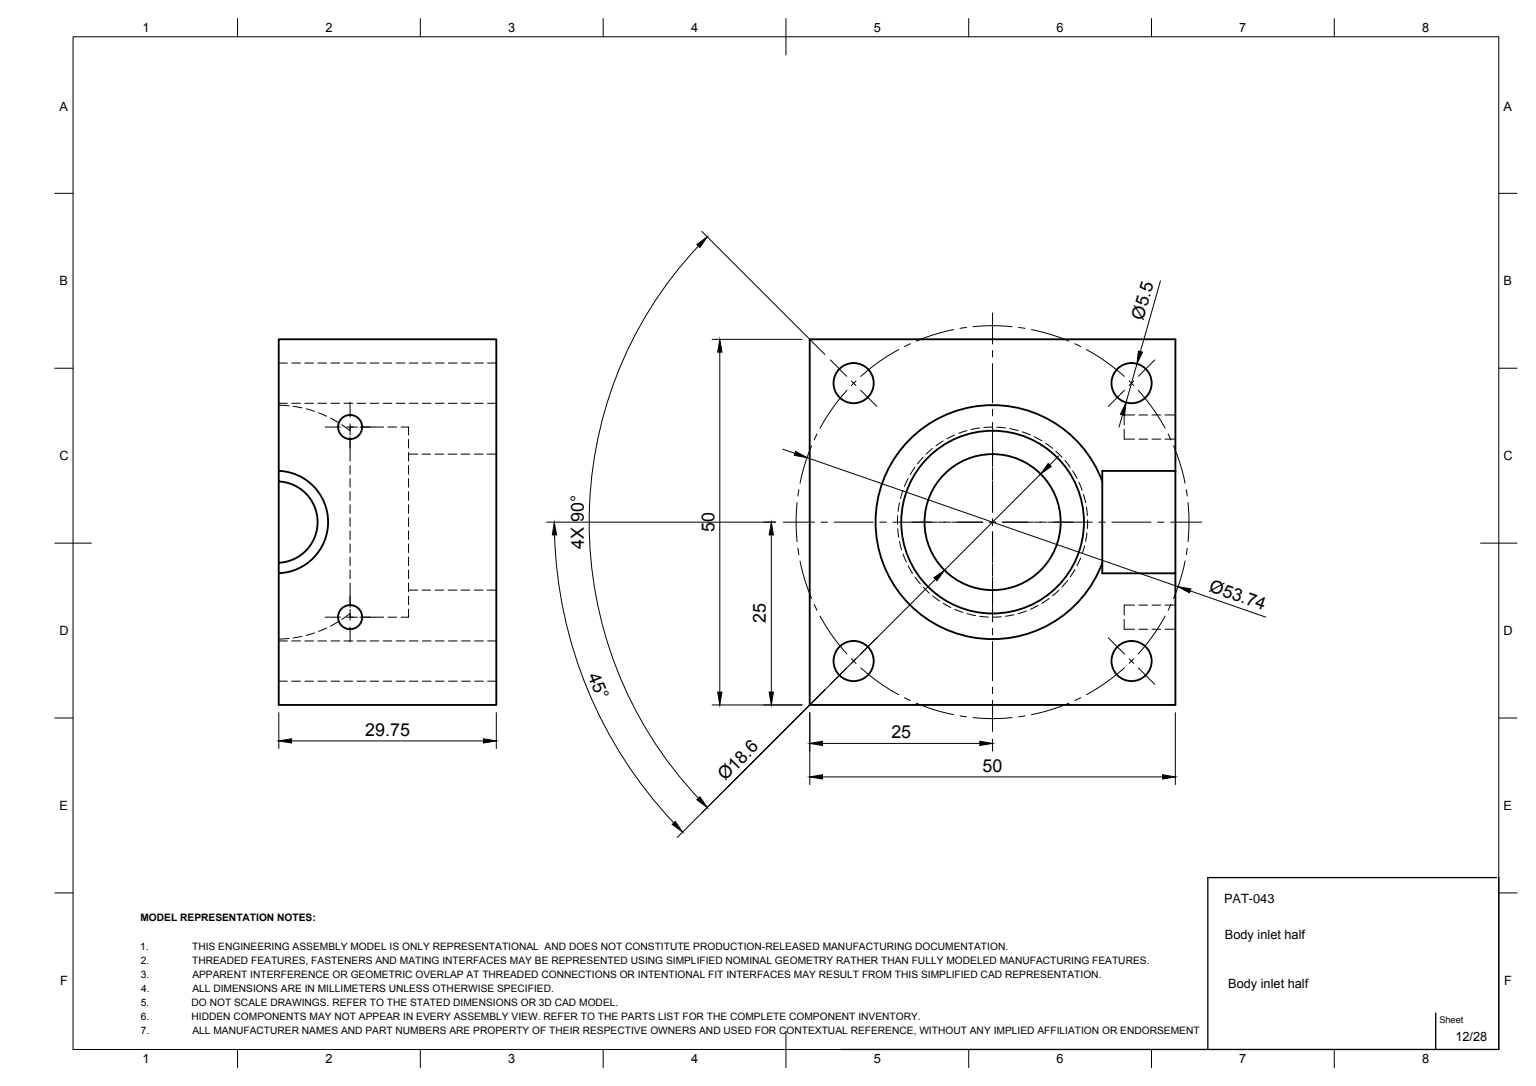
ISO-10303-21;
HEADER;
/* Generated by software containing ST-Developer
 * from STEP Tools, Inc. (www.steptools.com) 
 */

FILE_DESCRIPTION(
/* description */ ('Four-valve pipe header'),
/* implementation_level */ '2;1');

FILE_NAME(
/* name */ 'Body inlet half.step',
/* time_stamp */ '2026-10-29T16:56:19-07:00',
/* author */ (''),
/* organization */ (''),
/* preprocessor_version */ 'ST-DEVELOPER v20.2',
/* originating_system */ 'Autodesk Translation Framework v15.17.0.0',
/* authorisation */ '');

FILE_SCHEMA (('AUTOMOTIVE_DESIGN { 1 0 10303 214 3 1 1 }'));
ENDSEC;

DATA;
#10=MECHANICAL_DESIGN_GEOMETRIC_PRESENTATION_REPRESENTATION('',(#338),#10119);
#242=SPHERICAL_SURFACE('',#6142,1.6);
#286=SHAPE_REPRESENTATION_RELATIONSHIP('SRR','None',#10248,#312);
#312=ADVANCED_BREP_SHAPE_REPRESENTATION('',(#364),#10097);
#338=STYLED_ITEM('',(#10449),#364);
#364=MANIFOLD_SOLID_BREP('Body1',#5584);
#456=FACE_BOUND('',#1223,.T.);
#457=FACE_BOUND('',#1224,.T.);
#458=FACE_BOUND('',#1228,.T.);
#459=FACE_BOUND('',#1230,.T.);
#460=FACE_BOUND('',#1232,.T.);
#461=FACE_BOUND('',#1234,.T.);
#462=FACE_BOUND('',#1235,.T.);
#463=FACE_BOUND('',#1236,.T.);
#464=FACE_BOUND('',#1237,.T.);
#465=FACE_BOUND('',#1240,.T.);
#466=FACE_BOUND('',#1241,.T.);
#467=FACE_BOUND('',#1242,.T.);
#468=FACE_BOUND('',#1243,.T.);
#469=FACE_BOUND('',#1244,.T.);
#597=PLANE('',#6110);
#598=PLANE('',#6114);
#599=PLANE('',#6130);
#600=PLANE('',#6132);
#601=PLANE('',#6139);
#602=PLANE('',#6141);
#603=PLANE('',#6144);
#604=PLANE('',#6145);
#605=PLANE('',#6146);
#606=PLANE('',#6147);
#607=PLANE('',#6148);
#850=FACE_OUTER_BOUND('',#1212,.T.);
#851=FACE_OUTER_BOUND('',#1213,.T.);
#852=FACE_OUTER_BOUND('',#1214,.T.);
#853=FACE_OUTER_BOUND('',#1215,.T.);
#854=FACE_OUTER_BOUND('',#1216,.T.);
#855=FACE_OUTER_BOUND('',#1217,.T.);
#856=FACE_OUTER_BOUND('',#1218,.T.);
#857=FACE_OUTER_BOUND('',#1219,.T.);
#858=FACE_OUTER_BOUND('',#1220,.T.);
#859=FACE_OUTER_BOUND('',#1221,.T.);
#860=FACE_OUTER_BOUND('',#1222,.T.);
#861=FACE_OUTER_BOUND('',#1225,.T.);
#862=FACE_OUTER_BOUND('',#1226,.T.);
#863=FACE_OUTER_BOUND('',#1227,.T.);
#864=FACE_OUTER_BOUND('',#1229,.T.);
#865=FACE_OUTER_BOUND('',#1231,.T.);
#866=FACE_OUTER_BOUND('',#1233,.T.);
#867=FACE_OUTER_BOUND('',#1238,.T.);
#868=FACE_OUTER_BOUND('',#1239,.T.);
#869=FACE_OUTER_BOUND('',#1245,.T.);
#870=FACE_OUTER_BOUND('',#1246,.T.);
#1212=EDGE_LOOP('',(#4215,#4216,#4217,#4218));
#1213=EDGE_LOOP('',(#4219));
#1214=EDGE_LOOP('',(#4220,#4221,#4222,#4223));
#1215=EDGE_LOOP('',(#4224));
#1216=EDGE_LOOP('',(#4225,#4226,#4227,#4228));
#1217=EDGE_LOOP('',(#4229,#4230,#4231,#4232));
#1218=EDGE_LOOP('',(#4233,#4234,#4235,#4236));
#1219=EDGE_LOOP('',(#4237,#4238,#4239,#4240));
#1220=EDGE_LOOP('',(#4241,#4242,#4243,#4244));
#1221=EDGE_LOOP('',(#4245,#4246,#4247,#4248));
#1222=EDGE_LOOP('',(#4249,#4250,#4251,#4252,#4253,#4254));
#1223=EDGE_LOOP('',(#4255));
#1224=EDGE_LOOP('',(#4256));
#1225=EDGE_LOOP('',(#4257,#4258,#4259,#4260));
#1226=EDGE_LOOP('',(#4261,#4262,#4263,#4264));
#1227=EDGE_LOOP('',(#4265));
#1228=EDGE_LOOP('',(#4266));
#1229=EDGE_LOOP('',(#4267));
#1230=EDGE_LOOP('',(#4268));
#1231=EDGE_LOOP('',(#4269,#4270));
#1232=EDGE_LOOP('',(#4271));
#1233=EDGE_LOOP('',(#4272,#4273,#4274,#4275,#4276,#4277,#4278,#4279,#4280,
#4281));
#1234=EDGE_LOOP('',(#4282));
#1235=EDGE_LOOP('',(#4283));
#1236=EDGE_LOOP('',(#4284));
#1237=EDGE_LOOP('',(#4285));
#1238=EDGE_LOOP('',(#4286,#4287,#4288,#4289));
#1239=EDGE_LOOP('',(#4290,#4291,#4292,#4293));
#1240=EDGE_LOOP('',(#4294));
#1241=EDGE_LOOP('',(#4295));
#1242=EDGE_LOOP('',(#4296));
#1243=EDGE_LOOP('',(#4297));
#1244=EDGE_LOOP('',(#4298));
#1245=EDGE_LOOP('',(#4299,#4300,#4301,#4302));
#1246=EDGE_LOOP('',(#4303,#4304,#4305,#4306));
#1639=LINE('',#8960,#2057);
#1640=LINE('',#8967,#2058);
#1641=LINE('',#8974,#2059);
#1642=LINE('',#8980,#2060);
#1643=LINE('',#8986,#2061);
#1644=LINE('',#8992,#2062);
#1645=LINE('',#8997,#2063);
#1646=LINE('',#9001,#2064);
#1647=LINE('',#9005,#2065);
#1648=LINE('',#9008,#2066);
#1649=LINE('',#9011,#2067);
#1650=LINE('',#9013,#2068);
#1651=LINE('',#9015,#2069);
#1652=LINE('',#9017,#2070);
#1653=LINE('',#9018,#2071);
#1654=LINE('',#9023,#2072);
#1655=LINE('',#9029,#2073);
#1656=LINE('',#9039,#2074);
#1657=LINE('',#9041,#2075);
#1658=LINE('',#9042,#2076);
#1659=LINE('',#9045,#2077);
#1660=LINE('',#9046,#2078);
#1661=LINE('',#9049,#2079);
#1662=LINE('',#9050,#2080);
#1663=LINE('',#9052,#2081);
#2057=VECTOR('',#7116,0.165);
#2058=VECTOR('',#7125,0.165);
#2059=VECTOR('',#7134,0.275);
#2060=VECTOR('',#7141,0.275);
#2061=VECTOR('',#7148,0.275);
#2062=VECTOR('',#7155,0.275);
#2063=VECTOR('',#7160,1.);
#2064=VECTOR('',#7163,1.);
#2065=VECTOR('',#7168,1.);
#2066=VECTOR('',#7171,1.);
#2067=VECTOR('',#7174,1.);
#2068=VECTOR('',#7175,1.);
#2069=VECTOR('',#7176,1.);
#2070=VECTOR('',#7177,1.);
#2071=VECTOR('',#7178,1.);
#2072=VECTOR('',#7183,0.93);
#2073=VECTOR('',#7190,1.3);
#2074=VECTOR('',#7205,1.);
#2075=VECTOR('',#7206,1.);
#2076=VECTOR('',#7207,1.);
#2077=VECTOR('',#7210,1.);
#2078=VECTOR('',#7211,1.);
#2079=VECTOR('',#7214,1.);
#2080=VECTOR('',#7215,1.);
#2081=VECTOR('',#7218,1.);
#2424=CIRCLE('',#6108,0.165);
#2425=CIRCLE('',#6109,0.165);
#2426=CIRCLE('',#6112,0.165);
#2427=CIRCLE('',#6113,0.165);
#2428=CIRCLE('',#6116,0.275);
#2429=CIRCLE('',#6117,0.275);
#2430=CIRCLE('',#6119,0.275);
#2431=CIRCLE('',#6120,0.275);
#2432=CIRCLE('',#6122,0.275);
#2433=CIRCLE('',#6123,0.275);
#2434=CIRCLE('',#6125,0.275);
#2435=CIRCLE('',#6126,0.275);
#2436=CIRCLE('',#6128,0.7);
#2437=CIRCLE('',#6129,0.7);
#2438=CIRCLE('',#6131,0.556776436283003);
#2439=CIRCLE('',#6134,0.93);
#2440=CIRCLE('',#6135,0.93);
#2441=CIRCLE('',#6137,1.3);
#2442=CIRCLE('',#6138,1.3);
#2443=CIRCLE('',#6140,1.24899959967968);
#2444=CIRCLE('',#6143,1.59980467557762);
#2732=VERTEX_POINT('',#8957);
#2733=VERTEX_POINT('',#8959);
#2734=VERTEX_POINT('',#8964);
#2735=VERTEX_POINT('',#8966);
#2736=VERTEX_POINT('',#8971);
#2737=VERTEX_POINT('',#8973);
#2738=VERTEX_POINT('',#8977);
#2739=VERTEX_POINT('',#8979);
#2740=VERTEX_POINT('',#8983);
#2741=VERTEX_POINT('',#8985);
#2742=VERTEX_POINT('',#8989);
#2743=VERTEX_POINT('',#8991);
#2744=VERTEX_POINT('',#8995);
#2745=VERTEX_POINT('',#8996);
#2746=VERTEX_POINT('',#8998);
#2747=VERTEX_POINT('',#9000);
#2748=VERTEX_POINT('',#9004);
#2749=VERTEX_POINT('',#9006);
#2750=VERTEX_POINT('',#9010);
#2751=VERTEX_POINT('',#9012);
#2752=VERTEX_POINT('',#9014);
#2753=VERTEX_POINT('',#9016);
#2754=VERTEX_POINT('',#9020);
#2755=VERTEX_POINT('',#9022);
#2756=VERTEX_POINT('',#9026);
#2757=VERTEX_POINT('',#9028);
#2758=VERTEX_POINT('',#9032);
#2759=VERTEX_POINT('',#9038);
#2760=VERTEX_POINT('',#9040);
#2761=VERTEX_POINT('',#9044);
#2762=VERTEX_POINT('',#9048);
#3274=EDGE_CURVE('',#2732,#2732,#2424,.T.);
#3275=EDGE_CURVE('',#2732,#2733,#1639,.T.);
#3276=EDGE_CURVE('',#2733,#2733,#2425,.T.);
#3277=EDGE_CURVE('',#2734,#2734,#2426,.T.);
#3278=EDGE_CURVE('',#2734,#2735,#1640,.T.);
#3279=EDGE_CURVE('',#2735,#2735,#2427,.T.);
#3280=EDGE_CURVE('',#2736,#2736,#2428,.T.);
#3281=EDGE_CURVE('',#2736,#2737,#1641,.T.);
#3282=EDGE_CURVE('',#2737,#2737,#2429,.T.);
#3283=EDGE_CURVE('',#2738,#2738,#2430,.T.);
#3284=EDGE_CURVE('',#2738,#2739,#1642,.T.);
#3285=EDGE_CURVE('',#2739,#2739,#2431,.T.);
#3286=EDGE_CURVE('',#2740,#2740,#2432,.T.);
#3287=EDGE_CURVE('',#2740,#2741,#1643,.T.);
#3288=EDGE_CURVE('',#2741,#2741,#2433,.T.);
#3289=EDGE_CURVE('',#2742,#2742,#2434,.T.);
#3290=EDGE_CURVE('',#2742,#2743,#1644,.T.);
#3291=EDGE_CURVE('',#2743,#2743,#2435,.T.);
#3292=EDGE_CURVE('',#2744,#2745,#1645,.T.);
#3293=EDGE_CURVE('',#2746,#2744,#2436,.T.);
#3294=EDGE_CURVE('',#2747,#2746,#1646,.T.);
#3295=EDGE_CURVE('',#2745,#2747,#2437,.T.);
#3296=EDGE_CURVE('',#2748,#2744,#1647,.T.);
#3297=EDGE_CURVE('',#2749,#2748,#2438,.T.);
#3298=EDGE_CURVE('',#2746,#2749,#1648,.T.);
#3299=EDGE_CURVE('',#2747,#2750,#1649,.T.);
#3300=EDGE_CURVE('',#2750,#2751,#1650,.T.);
#3301=EDGE_CURVE('',#2751,#2752,#1651,.T.);
#3302=EDGE_CURVE('',#2752,#2753,#1652,.T.);
#3303=EDGE_CURVE('',#2753,#2745,#1653,.T.);
#3304=EDGE_CURVE('',#2754,#2754,#2439,.T.);
#3305=EDGE_CURVE('',#2754,#2755,#1654,.T.);
#3306=EDGE_CURVE('',#2755,#2755,#2440,.T.);
#3307=EDGE_CURVE('',#2756,#2756,#2441,.T.);
#3308=EDGE_CURVE('',#2756,#2757,#1655,.T.);
#3309=EDGE_CURVE('',#2757,#2757,#2442,.T.);
#3310=EDGE_CURVE('',#2758,#2758,#2443,.T.);
#3311=EDGE_CURVE('',#2749,#2748,#2444,.T.);
#3312=EDGE_CURVE('',#2759,#2753,#1656,.T.);
#3313=EDGE_CURVE('',#2759,#2760,#1657,.T.);
#3314=EDGE_CURVE('',#2760,#2750,#1658,.T.);
#3315=EDGE_CURVE('',#2761,#2759,#1659,.T.);
#3316=EDGE_CURVE('',#2761,#2752,#1660,.T.);
#3317=EDGE_CURVE('',#2762,#2761,#1661,.T.);
#3318=EDGE_CURVE('',#2762,#2751,#1662,.T.);
#3319=EDGE_CURVE('',#2760,#2762,#1663,.T.);
#4215=ORIENTED_EDGE('',*,*,#3274,.F.);
#4216=ORIENTED_EDGE('',*,*,#3275,.T.);
#4217=ORIENTED_EDGE('',*,*,#3276,.F.);
#4218=ORIENTED_EDGE('',*,*,#3275,.F.);
#4219=ORIENTED_EDGE('',*,*,#3274,.T.);
#4220=ORIENTED_EDGE('',*,*,#3277,.F.);
#4221=ORIENTED_EDGE('',*,*,#3278,.T.);
#4222=ORIENTED_EDGE('',*,*,#3279,.F.);
#4223=ORIENTED_EDGE('',*,*,#3278,.F.);
#4224=ORIENTED_EDGE('',*,*,#3277,.T.);
#4225=ORIENTED_EDGE('',*,*,#3280,.F.);
#4226=ORIENTED_EDGE('',*,*,#3281,.T.);
#4227=ORIENTED_EDGE('',*,*,#3282,.F.);
#4228=ORIENTED_EDGE('',*,*,#3281,.F.);
#4229=ORIENTED_EDGE('',*,*,#3283,.F.);
#4230=ORIENTED_EDGE('',*,*,#3284,.T.);
#4231=ORIENTED_EDGE('',*,*,#3285,.F.);
#4232=ORIENTED_EDGE('',*,*,#3284,.F.);
#4233=ORIENTED_EDGE('',*,*,#3286,.F.);
#4234=ORIENTED_EDGE('',*,*,#3287,.T.);
#4235=ORIENTED_EDGE('',*,*,#3288,.F.);
#4236=ORIENTED_EDGE('',*,*,#3287,.F.);
#4237=ORIENTED_EDGE('',*,*,#3289,.F.);
#4238=ORIENTED_EDGE('',*,*,#3290,.T.);
#4239=ORIENTED_EDGE('',*,*,#3291,.F.);
#4240=ORIENTED_EDGE('',*,*,#3290,.F.);
#4241=ORIENTED_EDGE('',*,*,#3292,.F.);
#4242=ORIENTED_EDGE('',*,*,#3293,.F.);
#4243=ORIENTED_EDGE('',*,*,#3294,.F.);
#4244=ORIENTED_EDGE('',*,*,#3295,.F.);
#4245=ORIENTED_EDGE('',*,*,#3296,.F.);
#4246=ORIENTED_EDGE('',*,*,#3297,.F.);
#4247=ORIENTED_EDGE('',*,*,#3298,.F.);
#4248=ORIENTED_EDGE('',*,*,#3293,.T.);
#4249=ORIENTED_EDGE('',*,*,#3295,.T.);
#4250=ORIENTED_EDGE('',*,*,#3299,.T.);
#4251=ORIENTED_EDGE('',*,*,#3300,.T.);
#4252=ORIENTED_EDGE('',*,*,#3301,.T.);
#4253=ORIENTED_EDGE('',*,*,#3302,.T.);
#4254=ORIENTED_EDGE('',*,*,#3303,.T.);
#4255=ORIENTED_EDGE('',*,*,#3276,.T.);
#4256=ORIENTED_EDGE('',*,*,#3279,.T.);
#4257=ORIENTED_EDGE('',*,*,#3304,.F.);
#4258=ORIENTED_EDGE('',*,*,#3305,.T.);
#4259=ORIENTED_EDGE('',*,*,#3306,.F.);
#4260=ORIENTED_EDGE('',*,*,#3305,.F.);
#4261=ORIENTED_EDGE('',*,*,#3307,.F.);
#4262=ORIENTED_EDGE('',*,*,#3308,.T.);
#4263=ORIENTED_EDGE('',*,*,#3309,.T.);
#4264=ORIENTED_EDGE('',*,*,#3308,.F.);
#4265=ORIENTED_EDGE('',*,*,#3309,.F.);
#4266=ORIENTED_EDGE('',*,*,#3310,.F.);
#4267=ORIENTED_EDGE('',*,*,#3307,.T.);
#4268=ORIENTED_EDGE('',*,*,#3306,.T.);
#4269=ORIENTED_EDGE('',*,*,#3297,.T.);
#4270=ORIENTED_EDGE('',*,*,#3311,.F.);
#4271=ORIENTED_EDGE('',*,*,#3310,.T.);
#4272=ORIENTED_EDGE('',*,*,#3292,.T.);
#4273=ORIENTED_EDGE('',*,*,#3303,.F.);
#4274=ORIENTED_EDGE('',*,*,#3312,.F.);
#4275=ORIENTED_EDGE('',*,*,#3313,.T.);
#4276=ORIENTED_EDGE('',*,*,#3314,.T.);
#4277=ORIENTED_EDGE('',*,*,#3299,.F.);
#4278=ORIENTED_EDGE('',*,*,#3294,.T.);
#4279=ORIENTED_EDGE('',*,*,#3298,.T.);
#4280=ORIENTED_EDGE('',*,*,#3311,.T.);
#4281=ORIENTED_EDGE('',*,*,#3296,.T.);
#4282=ORIENTED_EDGE('',*,*,#3282,.T.);
#4283=ORIENTED_EDGE('',*,*,#3285,.T.);
#4284=ORIENTED_EDGE('',*,*,#3288,.T.);
#4285=ORIENTED_EDGE('',*,*,#3291,.T.);
#4286=ORIENTED_EDGE('',*,*,#3315,.T.);
#4287=ORIENTED_EDGE('',*,*,#3312,.T.);
#4288=ORIENTED_EDGE('',*,*,#3302,.F.);
#4289=ORIENTED_EDGE('',*,*,#3316,.F.);
#4290=ORIENTED_EDGE('',*,*,#3317,.T.);
#4291=ORIENTED_EDGE('',*,*,#3316,.T.);
#4292=ORIENTED_EDGE('',*,*,#3301,.F.);
#4293=ORIENTED_EDGE('',*,*,#3318,.F.);
#4294=ORIENTED_EDGE('',*,*,#3304,.T.);
#4295=ORIENTED_EDGE('',*,*,#3289,.T.);
#4296=ORIENTED_EDGE('',*,*,#3286,.T.);
#4297=ORIENTED_EDGE('',*,*,#3283,.T.);
#4298=ORIENTED_EDGE('',*,*,#3280,.T.);
#4299=ORIENTED_EDGE('',*,*,#3319,.T.);
#4300=ORIENTED_EDGE('',*,*,#3318,.T.);
#4301=ORIENTED_EDGE('',*,*,#3300,.F.);
#4302=ORIENTED_EDGE('',*,*,#3314,.F.);
#4303=ORIENTED_EDGE('',*,*,#3319,.F.);
#4304=ORIENTED_EDGE('',*,*,#3313,.F.);
#4305=ORIENTED_EDGE('',*,*,#3315,.F.);
#4306=ORIENTED_EDGE('',*,*,#3317,.F.);
#5188=CYLINDRICAL_SURFACE('',#6107,0.165);
#5189=CYLINDRICAL_SURFACE('',#6111,0.165);
#5190=CYLINDRICAL_SURFACE('',#6115,0.275);
#5191=CYLINDRICAL_SURFACE('',#6118,0.275);
#5192=CYLINDRICAL_SURFACE('',#6121,0.275);
#5193=CYLINDRICAL_SURFACE('',#6124,0.275);
#5194=CYLINDRICAL_SURFACE('',#6127,0.7);
#5195=CYLINDRICAL_SURFACE('',#6133,0.93);
#5196=CYLINDRICAL_SURFACE('',#6136,1.3);
#5350=ADVANCED_FACE('',(#850),#5188,.F.);
#5351=ADVANCED_FACE('',(#851),#597,.T.);
#5352=ADVANCED_FACE('',(#852),#5189,.F.);
#5353=ADVANCED_FACE('',(#853),#598,.T.);
#5354=ADVANCED_FACE('',(#854),#5190,.F.);
#5355=ADVANCED_FACE('',(#855),#5191,.F.);
#5356=ADVANCED_FACE('',(#856),#5192,.F.);
#5357=ADVANCED_FACE('',(#857),#5193,.F.);
#5358=ADVANCED_FACE('',(#858),#5194,.F.);
#5359=ADVANCED_FACE('',(#859),#599,.T.);
#5360=ADVANCED_FACE('',(#860,#456,#457),#600,.T.);
#5361=ADVANCED_FACE('',(#861),#5195,.F.);
#5362=ADVANCED_FACE('',(#862),#5196,.F.);
#5363=ADVANCED_FACE('',(#863,#458),#601,.F.);
#5364=ADVANCED_FACE('',(#864,#459),#602,.T.);
#5365=ADVANCED_FACE('',(#865,#460),#242,.F.);
#5366=ADVANCED_FACE('',(#866,#461,#462,#463,#464),#603,.T.);
#5367=ADVANCED_FACE('',(#867),#604,.T.);
#5368=ADVANCED_FACE('',(#868,#465,#466,#467,#468,#469),#605,.T.);
#5369=ADVANCED_FACE('',(#869),#606,.T.);
#5370=ADVANCED_FACE('',(#870),#607,.F.);
#5584=CLOSED_SHELL('',(#5350,#5351,#5352,#5353,#5354,#5355,#5356,#5357,
#5358,#5359,#5360,#5361,#5362,#5363,#5364,#5365,#5366,#5367,#5368,#5369,
#5370));
#6106=AXIS2_PLACEMENT_3D('',#8955,#7110,#7111);
#6107=AXIS2_PLACEMENT_3D('',#8956,#7112,#7113);
#6108=AXIS2_PLACEMENT_3D('',#8958,#7114,#7115);
#6109=AXIS2_PLACEMENT_3D('',#8961,#7117,#7118);
#6110=AXIS2_PLACEMENT_3D('',#8962,#7119,#7120);
#6111=AXIS2_PLACEMENT_3D('',#8963,#7121,#7122);
#6112=AXIS2_PLACEMENT_3D('',#8965,#7123,#7124);
#6113=AXIS2_PLACEMENT_3D('',#8968,#7126,#7127);
#6114=AXIS2_PLACEMENT_3D('',#8969,#7128,#7129);
#6115=AXIS2_PLACEMENT_3D('',#8970,#7130,#7131);
#6116=AXIS2_PLACEMENT_3D('',#8972,#7132,#7133);
#6117=AXIS2_PLACEMENT_3D('',#8975,#7135,#7136);
#6118=AXIS2_PLACEMENT_3D('',#8976,#7137,#7138);
#6119=AXIS2_PLACEMENT_3D('',#8978,#7139,#7140);
#6120=AXIS2_PLACEMENT_3D('',#8981,#7142,#7143);
#6121=AXIS2_PLACEMENT_3D('',#8982,#7144,#7145);
#6122=AXIS2_PLACEMENT_3D('',#8984,#7146,#7147);
#6123=AXIS2_PLACEMENT_3D('',#8987,#7149,#7150);
#6124=AXIS2_PLACEMENT_3D('',#8988,#7151,#7152);
#6125=AXIS2_PLACEMENT_3D('',#8990,#7153,#7154);
#6126=AXIS2_PLACEMENT_3D('',#8993,#7156,#7157);
#6127=AXIS2_PLACEMENT_3D('',#8994,#7158,#7159);
#6128=AXIS2_PLACEMENT_3D('',#8999,#7161,#7162);
#6129=AXIS2_PLACEMENT_3D('',#9002,#7164,#7165);
#6130=AXIS2_PLACEMENT_3D('',#9003,#7166,#7167);
#6131=AXIS2_PLACEMENT_3D('',#9007,#7169,#7170);
#6132=AXIS2_PLACEMENT_3D('',#9009,#7172,#7173);
#6133=AXIS2_PLACEMENT_3D('',#9019,#7179,#7180);
#6134=AXIS2_PLACEMENT_3D('',#9021,#7181,#7182);
#6135=AXIS2_PLACEMENT_3D('',#9024,#7184,#7185);
#6136=AXIS2_PLACEMENT_3D('',#9025,#7186,#7187);
#6137=AXIS2_PLACEMENT_3D('',#9027,#7188,#7189);
#6138=AXIS2_PLACEMENT_3D('',#9030,#7191,#7192);
#6139=AXIS2_PLACEMENT_3D('',#9031,#7193,#7194);
#6140=AXIS2_PLACEMENT_3D('',#9033,#7195,#7196);
#6141=AXIS2_PLACEMENT_3D('',#9034,#7197,#7198);
#6142=AXIS2_PLACEMENT_3D('',#9035,#7199,#7200);
#6143=AXIS2_PLACEMENT_3D('',#9036,#7201,#7202);
#6144=AXIS2_PLACEMENT_3D('',#9037,#7203,#7204);
#6145=AXIS2_PLACEMENT_3D('',#9043,#7208,#7209);
#6146=AXIS2_PLACEMENT_3D('',#9047,#7212,#7213);
#6147=AXIS2_PLACEMENT_3D('',#9051,#7216,#7217);
#6148=AXIS2_PLACEMENT_3D('',#9053,#7219,#7220);
#7110=DIRECTION('axis',(0.,0.,1.));
#7111=DIRECTION('refdir',(1.,0.,0.));
#7112=DIRECTION('center_axis',(0.,0.,1.));
#7113=DIRECTION('ref_axis',(1.,0.,0.));
#7114=DIRECTION('center_axis',(0.,0.,1.));
#7115=DIRECTION('ref_axis',(1.,0.,0.));
#7116=DIRECTION('',(0.,0.,1.));
#7117=DIRECTION('center_axis',(0.,0.,-1.));
#7118=DIRECTION('ref_axis',(1.,0.,0.));
#7119=DIRECTION('center_axis',(0.,0.,1.));
#7120=DIRECTION('ref_axis',(1.,0.,0.));
#7121=DIRECTION('center_axis',(0.,0.,1.));
#7122=DIRECTION('ref_axis',(1.,0.,0.));
#7123=DIRECTION('center_axis',(0.,0.,1.));
#7124=DIRECTION('ref_axis',(1.,0.,0.));
#7125=DIRECTION('',(0.,0.,1.));
#7126=DIRECTION('center_axis',(0.,0.,-1.));
#7127=DIRECTION('ref_axis',(1.,0.,0.));
#7128=DIRECTION('center_axis',(0.,0.,1.));
#7129=DIRECTION('ref_axis',(1.,0.,0.));
#7130=DIRECTION('center_axis',(0.,1.,0.));
#7131=DIRECTION('ref_axis',(1.,0.,0.));
#7132=DIRECTION('center_axis',(0.,1.,0.));
#7133=DIRECTION('ref_axis',(1.,0.,0.));
#7134=DIRECTION('',(0.,1.,0.));
#7135=DIRECTION('center_axis',(0.,-1.,0.));
#7136=DIRECTION('ref_axis',(1.,0.,0.));
#7137=DIRECTION('center_axis',(0.,1.,0.));
#7138=DIRECTION('ref_axis',(1.,0.,0.));
#7139=DIRECTION('center_axis',(0.,1.,0.));
#7140=DIRECTION('ref_axis',(1.,0.,0.));
#7141=DIRECTION('',(0.,1.,0.));
#7142=DIRECTION('center_axis',(0.,-1.,0.));
#7143=DIRECTION('ref_axis',(1.,0.,0.));
#7144=DIRECTION('center_axis',(0.,1.,0.));
#7145=DIRECTION('ref_axis',(1.,0.,0.));
#7146=DIRECTION('center_axis',(0.,1.,0.));
#7147=DIRECTION('ref_axis',(1.,0.,0.));
#7148=DIRECTION('',(0.,1.,0.));
#7149=DIRECTION('center_axis',(0.,-1.,0.));
#7150=DIRECTION('ref_axis',(1.,0.,0.));
#7151=DIRECTION('center_axis',(0.,1.,0.));
#7152=DIRECTION('ref_axis',(1.,0.,0.));
#7153=DIRECTION('center_axis',(0.,1.,0.));
#7154=DIRECTION('ref_axis',(1.,0.,0.));
#7155=DIRECTION('',(0.,1.,0.));
#7156=DIRECTION('center_axis',(0.,-1.,0.));
#7157=DIRECTION('ref_axis',(1.,0.,0.));
#7158=DIRECTION('center_axis',(0.,0.,1.));
#7159=DIRECTION('ref_axis',(1.,0.,0.));
#7160=DIRECTION('',(0.,0.,1.));
#7161=DIRECTION('center_axis',(0.,0.,1.));
#7162=DIRECTION('ref_axis',(1.,0.,0.));
#7163=DIRECTION('',(0.,0.,-1.));
#7164=DIRECTION('center_axis',(0.,0.,-1.));
#7165=DIRECTION('ref_axis',(1.,0.,0.));
#7166=DIRECTION('center_axis',(0.,0.,1.));
#7167=DIRECTION('ref_axis',(1.,0.,0.));
#7168=DIRECTION('',(1.,0.,0.));
#7169=DIRECTION('center_axis',(0.,0.,1.));
#7170=DIRECTION('ref_axis',(0.,-1.,0.));
#7171=DIRECTION('',(1.,0.,0.));
#7172=DIRECTION('center_axis',(0.,0.,1.));
#7173=DIRECTION('ref_axis',(1.,0.,0.));
#7174=DIRECTION('',(-1.,0.,0.));
#7175=DIRECTION('',(0.,-1.,0.));
#7176=DIRECTION('',(1.,0.,0.));
#7177=DIRECTION('',(0.,1.,0.));
#7178=DIRECTION('',(-1.,0.,0.));
#7179=DIRECTION('center_axis',(0.,1.,0.));
#7180=DIRECTION('ref_axis',(1.,0.,0.));
#7181=DIRECTION('center_axis',(0.,1.,0.));
#7182=DIRECTION('ref_axis',(1.,0.,0.));
#7183=DIRECTION('',(0.,1.,0.));
#7184=DIRECTION('center_axis',(0.,-1.,0.));
#7185=DIRECTION('ref_axis',(1.,0.,0.));
#7186=DIRECTION('center_axis',(0.,1.,0.));
#7187=DIRECTION('ref_axis',(1.,0.,0.));
#7188=DIRECTION('center_axis',(0.,1.,0.));
#7189=DIRECTION('ref_axis',(1.,0.,0.));
#7190=DIRECTION('',(0.,1.,0.));
#7191=DIRECTION('center_axis',(0.,1.,0.));
#7192=DIRECTION('ref_axis',(1.,0.,0.));
#7193=DIRECTION('center_axis',(0.,1.,0.));
#7194=DIRECTION('ref_axis',(1.,0.,0.));
#7195=DIRECTION('center_axis',(0.,-1.,0.));
#7196=DIRECTION('ref_axis',(0.,0.,-1.));
#7197=DIRECTION('center_axis',(0.,1.,0.));
#7198=DIRECTION('ref_axis',(1.,0.,0.));
#7199=DIRECTION('center_axis',(6.12323399573677E-17,0.,1.));
#7200=DIRECTION('ref_axis',(1.,0.,0.));
#7201=DIRECTION('center_axis',(0.,-1.,0.));
#7202=DIRECTION('ref_axis',(0.,0.,-1.));
#7203=DIRECTION('center_axis',(0.,1.,0.));
#7204=DIRECTION('ref_axis',(-1.,0.,0.));
#7205=DIRECTION('',(0.,0.,1.));
#7206=DIRECTION('',(-1.,0.,0.));
#7207=DIRECTION('',(0.,0.,1.));
#7208=DIRECTION('center_axis',(1.,0.,0.));
#7209=DIRECTION('ref_axis',(0.,1.,0.));
#7210=DIRECTION('',(0.,1.,0.));
#7211=DIRECTION('',(0.,0.,1.));
#7212=DIRECTION('center_axis',(0.,-1.,0.));
#7213=DIRECTION('ref_axis',(1.,0.,0.));
#7214=DIRECTION('',(1.,0.,0.));
#7215=DIRECTION('',(0.,0.,1.));
#7216=DIRECTION('center_axis',(-1.,0.,0.));
#7217=DIRECTION('ref_axis',(0.,-1.,0.));
#7218=DIRECTION('',(0.,-1.,0.));
#7219=DIRECTION('center_axis',(0.,0.,1.));
#7220=DIRECTION('ref_axis',(1.,0.,0.));
#8955=CARTESIAN_POINT('',(0.,0.,0.));
#8956=CARTESIAN_POINT('Origin',(-1.3,-1.,6.8));
#8957=CARTESIAN_POINT('',(-1.465,-1.,6.8));
#8958=CARTESIAN_POINT('Origin',(-1.3,-1.,6.8));
#8959=CARTESIAN_POINT('',(-1.465,-1.,7.5));
#8960=CARTESIAN_POINT('',(-1.465,-1.,6.8));
#8961=CARTESIAN_POINT('Origin',(-1.3,-1.,7.5));
#8962=CARTESIAN_POINT('Origin',(-1.3,-1.,6.8));
#8963=CARTESIAN_POINT('Origin',(1.3,-1.,6.8));
#8964=CARTESIAN_POINT('',(1.135,-1.,6.8));
#8965=CARTESIAN_POINT('Origin',(1.3,-1.,6.8));
#8966=CARTESIAN_POINT('',(1.135,-1.,7.5));
#8967=CARTESIAN_POINT('',(1.135,-1.,6.8));
#8968=CARTESIAN_POINT('Origin',(1.3,-1.,7.5));
#8969=CARTESIAN_POINT('Origin',(1.3,-1.,6.8));
#8970=CARTESIAN_POINT('Origin',(1.9,-3.1,3.1));
#8971=CARTESIAN_POINT('',(1.625,-3.,3.1));
#8972=CARTESIAN_POINT('Origin',(1.9,-3.,3.1));
#8973=CARTESIAN_POINT('',(1.625,-0.0249999999999999,3.1));
#8974=CARTESIAN_POINT('',(1.625,-3.1,3.1));
#8975=CARTESIAN_POINT('Origin',(1.9,-0.0249999999999999,3.1));
#8976=CARTESIAN_POINT('Origin',(-1.9,-3.1,6.9));
#8977=CARTESIAN_POINT('',(-2.175,-3.,6.9));
#8978=CARTESIAN_POINT('Origin',(-1.9,-3.,6.9));
#8979=CARTESIAN_POINT('',(-2.175,-0.0249999999999999,6.9));
#8980=CARTESIAN_POINT('',(-2.175,-3.1,6.9));
#8981=CARTESIAN_POINT('Origin',(-1.9,-0.0249999999999999,6.9));
#8982=CARTESIAN_POINT('Origin',(-1.9,-3.1,3.1));
#8983=CARTESIAN_POINT('',(-2.175,-3.,3.1));
#8984=CARTESIAN_POINT('Origin',(-1.9,-3.,3.1));
#8985=CARTESIAN_POINT('',(-2.175,-0.0249999999999999,3.1));
#8986=CARTESIAN_POINT('',(-2.175,-3.1,3.1));
#8987=CARTESIAN_POINT('Origin',(-1.9,-0.0249999999999999,3.1));
#8988=CARTESIAN_POINT('Origin',(1.9,-3.1,6.9));
#8989=CARTESIAN_POINT('',(1.625,-3.,6.9));
#8990=CARTESIAN_POINT('Origin',(1.9,-3.,6.9));
#8991=CARTESIAN_POINT('',(1.625,-0.0249999999999999,6.9));
#8992=CARTESIAN_POINT('',(1.625,-3.1,6.9));
#8993=CARTESIAN_POINT('Origin',(1.9,-0.0249999999999999,6.9));
#8994=CARTESIAN_POINT('Origin',(0.,0.,6.5));
#8995=CARTESIAN_POINT('',(0.699553428981661,-0.025,6.5));
#8996=CARTESIAN_POINT('',(0.699553428981661,-0.025,7.5));
#8997=CARTESIAN_POINT('',(0.699553428981661,-0.025,6.5));
#8998=CARTESIAN_POINT('',(-0.699553428981661,-0.025,6.5));
#8999=CARTESIAN_POINT('Origin',(0.,0.,6.5));
#9000=CARTESIAN_POINT('',(-0.699553428981661,-0.025,7.5));
#9001=CARTESIAN_POINT('',(-0.699553428981661,-0.025,6.5));
#9002=CARTESIAN_POINT('Origin',(0.,0.,7.5));
#9003=CARTESIAN_POINT('Origin',(0.,0.,6.5));
#9004=CARTESIAN_POINT('',(0.556214886532175,-0.025,6.5));
#9005=CARTESIAN_POINT('',(1.25,-0.025,6.5));
#9006=CARTESIAN_POINT('',(-0.556214886532175,-0.025,6.5));
#9007=CARTESIAN_POINT('Origin',(0.,0.,6.5));
#9008=CARTESIAN_POINT('',(1.25,-0.025,6.5));
#9009=CARTESIAN_POINT('Origin',(0.,-1.5125,7.5));
#9010=CARTESIAN_POINT('',(-2.5,-0.025,7.5));
#9011=CARTESIAN_POINT('',(2.5,-0.025,7.5));
#9012=CARTESIAN_POINT('',(-2.5,-3.,7.5));
#9013=CARTESIAN_POINT('',(-2.5,-0.025,7.5));
#9014=CARTESIAN_POINT('',(2.5,-3.,7.5));
#9015=CARTESIAN_POINT('',(-2.5,-3.,7.5));
#9016=CARTESIAN_POINT('',(2.5,-0.025,7.5));
#9017=CARTESIAN_POINT('',(2.5,-3.,7.5));
#9018=CARTESIAN_POINT('',(2.5,-0.025,7.5));
#9019=CARTESIAN_POINT('Origin',(0.,-3.1,5.));
#9020=CARTESIAN_POINT('',(-0.93,-3.,5.));
#9021=CARTESIAN_POINT('Origin',(0.,-3.,5.));
#9022=CARTESIAN_POINT('',(-0.93,-1.8,5.));
#9023=CARTESIAN_POINT('',(-0.93,-3.1,5.));
#9024=CARTESIAN_POINT('Origin',(0.,-1.8,5.));
#9025=CARTESIAN_POINT('Origin',(0.,-1.8,5.));
#9026=CARTESIAN_POINT('',(-1.3,-1.8,5.));
#9027=CARTESIAN_POINT('Origin',(0.,-1.8,5.));
#9028=CARTESIAN_POINT('',(-1.3,-1.,5.));
#9029=CARTESIAN_POINT('',(-1.3,-1.8,5.));
#9030=CARTESIAN_POINT('Origin',(0.,-1.,5.));
#9031=CARTESIAN_POINT('Origin',(0.,-1.,5.));
#9032=CARTESIAN_POINT('',(-1.52958336188405E-16,-1.,6.24899959967968));
#9033=CARTESIAN_POINT('Origin',(0.,-1.,5.));
#9034=CARTESIAN_POINT('Origin',(0.,-1.8,5.));
#9035=CARTESIAN_POINT('Origin',(0.,0.,5.));
#9036=CARTESIAN_POINT('Origin',(0.,-0.025,5.));
#9037=CARTESIAN_POINT('Origin',(2.5,-0.025,2.5));
#9038=CARTESIAN_POINT('',(2.5,-0.025,2.5));
#9039=CARTESIAN_POINT('',(2.5,-0.025,2.5));
#9040=CARTESIAN_POINT('',(-2.5,-0.025,2.5));
#9041=CARTESIAN_POINT('',(2.5,-0.025,2.5));
#9042=CARTESIAN_POINT('',(-2.5,-0.025,2.5));
#9043=CARTESIAN_POINT('Origin',(2.5,-3.,2.5));
#9044=CARTESIAN_POINT('',(2.5,-3.,2.5));
#9045=CARTESIAN_POINT('',(2.5,-3.,2.5));
#9046=CARTESIAN_POINT('',(2.5,-3.,2.5));
#9047=CARTESIAN_POINT('Origin',(-2.5,-3.,2.5));
#9048=CARTESIAN_POINT('',(-2.5,-3.,2.5));
#9049=CARTESIAN_POINT('',(-2.5,-3.,2.5));
#9050=CARTESIAN_POINT('',(-2.5,-3.,2.5));
#9051=CARTESIAN_POINT('Origin',(-2.5,-0.025,2.5));
#9052=CARTESIAN_POINT('',(-2.5,-0.025,2.5));
#9053=CARTESIAN_POINT('Origin',(0.,-1.5125,2.5));
#10066=UNCERTAINTY_MEASURE_WITH_UNIT(LENGTH_MEASURE(0.001),#10120,
'DISTANCE_ACCURACY_VALUE',
'Maximum model space distance between geometric entities at asserted c
onnectivities');
#10088=UNCERTAINTY_MEASURE_WITH_UNIT(LENGTH_MEASURE(0.001),#10120,
'DISTANCE_ACCURACY_VALUE',
'Maximum model space distance between geometric entities at asserted c
onnectivities');
#10097=(
GEOMETRIC_REPRESENTATION_CONTEXT(3)
GLOBAL_UNCERTAINTY_ASSIGNED_CONTEXT((#10066))
GLOBAL_UNIT_ASSIGNED_CONTEXT((#10120,#10122,#10123))
REPRESENTATION_CONTEXT('','3D')
);
#10119=(
GEOMETRIC_REPRESENTATION_CONTEXT(3)
GLOBAL_UNCERTAINTY_ASSIGNED_CONTEXT((#10088))
GLOBAL_UNIT_ASSIGNED_CONTEXT((#10120,#10122,#10123))
REPRESENTATION_CONTEXT('','3D')
);
#10120=(
LENGTH_UNIT()
NAMED_UNIT(*)
SI_UNIT(.CENTI.,.METRE.)
);
#10122=(
NAMED_UNIT(*)
PLANE_ANGLE_UNIT()
SI_UNIT($,.RADIAN.)
);
#10123=(
NAMED_UNIT(*)
SI_UNIT($,.STERADIAN.)
SOLID_ANGLE_UNIT()
);
#10132=SHAPE_DEFINITION_REPRESENTATION(#10162,#10248);
#10162=PRODUCT_DEFINITION_SHAPE('',$,#10279);
#10248=SHAPE_REPRESENTATION('',(#6106),#10097);
#10270=PRODUCT_DEFINITION_CONTEXT('part definition',#10362,'design');
#10279=PRODUCT_DEFINITION('Body inlet half','Body inlet half',#10309,#10270);
#10309=PRODUCT_DEFINITION_FORMATION('',$,#10372);
#10362=APPLICATION_CONTEXT(
'Core Data for Automotive Mechanical Design Process');
#10363=PRODUCT_CONTEXT('part definition',#10362,'mechanical');
#10372=PRODUCT('Body inlet half','Body inlet half','Body inlet half',(#10363));
#10443=COLOUR_RGB('Dark Blue',0.08,0.2,0.34);
#10444=FILL_AREA_STYLE_COLOUR('',#10443);
#10445=FILL_AREA_STYLE('',(#10444));
#10446=SURFACE_STYLE_FILL_AREA(#10445);
#10447=SURFACE_SIDE_STYLE('',(#10446));
#10448=SURFACE_STYLE_USAGE(.BOTH.,#10447);
#10449=PRESENTATION_STYLE_ASSIGNMENT((#10448));
ENDSEC;
END-ISO-10303-21;
